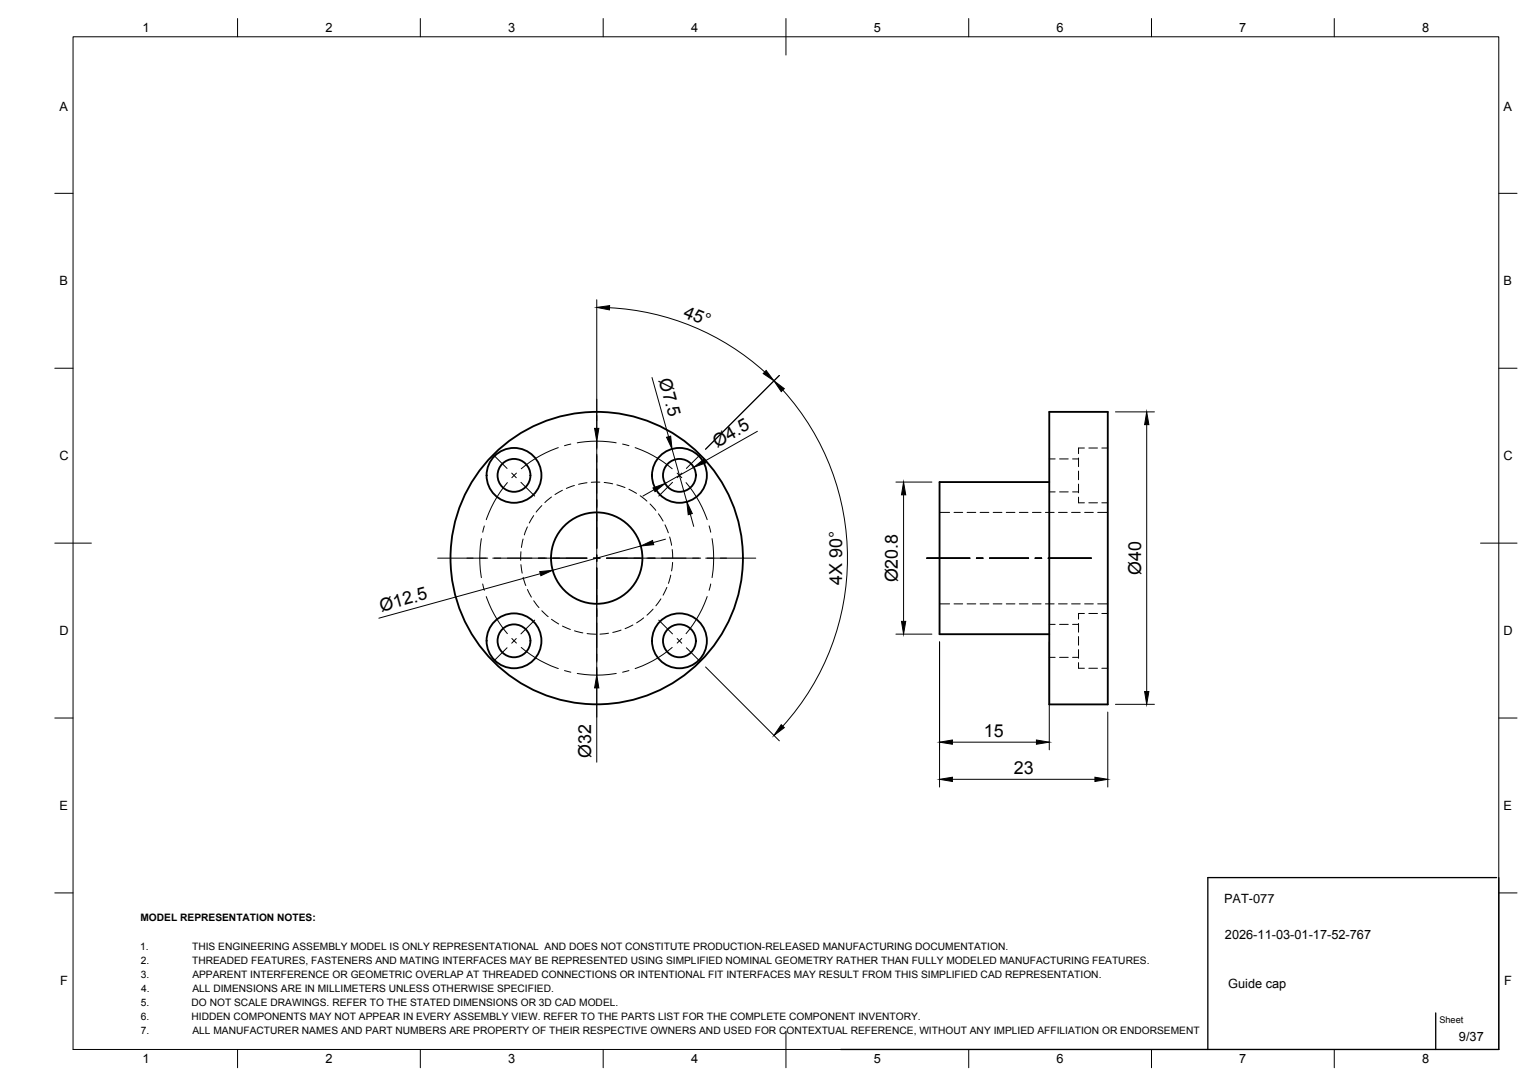
ISO-10303-21;
HEADER;
/* Generated by software containing ST-Developer
 * from STEP Tools, Inc. (www.steptools.com) 
 */

FILE_DESCRIPTION(
/* description */ ('Pallet stop with pneumatic fitting'),
/* implementation_level */ '2;1');

FILE_NAME(
/* name */ 'Guide cap.step',
/* time_stamp */ '2026-10-27T10:51:41-07:00',
/* author */ (''),
/* organization */ (''),
/* preprocessor_version */ 'ST-DEVELOPER v20.2',
/* originating_system */ 'Autodesk Translation Framework v15.17.0.0',
/* authorisation */ '');

FILE_SCHEMA (('AUTOMOTIVE_DESIGN { 1 0 10303 214 3 1 1 }'));
ENDSEC;

DATA;
#10=MECHANICAL_DESIGN_GEOMETRIC_PRESENTATION_REPRESENTATION('',(#361),#10265);
#297=SHAPE_REPRESENTATION_RELATIONSHIP('SRR','None',#10410,#329);
#329=ADVANCED_BREP_SHAPE_REPRESENTATION('',(#393),#10234);
#361=STYLED_ITEM('',(#10641),#393);
#393=MANIFOLD_SOLID_BREP('Body1',#5049);
#448=FACE_BOUND('',#1133,.T.);
#449=FACE_BOUND('',#1136,.T.);
#450=FACE_BOUND('',#1139,.T.);
#451=FACE_BOUND('',#1142,.T.);
#452=FACE_BOUND('',#1149,.T.);
#453=FACE_BOUND('',#1153,.T.);
#454=FACE_BOUND('',#1154,.T.);
#455=FACE_BOUND('',#1155,.T.);
#456=FACE_BOUND('',#1156,.T.);
#457=FACE_BOUND('',#1157,.T.);
#458=FACE_BOUND('',#1159,.T.);
#459=FACE_BOUND('',#1160,.T.);
#460=FACE_BOUND('',#1161,.T.);
#461=FACE_BOUND('',#1162,.T.);
#462=FACE_BOUND('',#1163,.T.);
#578=PLANE('',#5532);
#579=PLANE('',#5537);
#580=PLANE('',#5542);
#581=PLANE('',#5547);
#582=PLANE('',#5560);
#583=PLANE('',#5567);
#584=PLANE('',#5568);
#788=FACE_OUTER_BOUND('',#1131,.T.);
#789=FACE_OUTER_BOUND('',#1132,.T.);
#790=FACE_OUTER_BOUND('',#1134,.T.);
#791=FACE_OUTER_BOUND('',#1135,.T.);
#792=FACE_OUTER_BOUND('',#1137,.T.);
#793=FACE_OUTER_BOUND('',#1138,.T.);
#794=FACE_OUTER_BOUND('',#1140,.T.);
#795=FACE_OUTER_BOUND('',#1141,.T.);
#796=FACE_OUTER_BOUND('',#1143,.T.);
#797=FACE_OUTER_BOUND('',#1144,.T.);
#798=FACE_OUTER_BOUND('',#1145,.T.);
#799=FACE_OUTER_BOUND('',#1146,.T.);
#800=FACE_OUTER_BOUND('',#1147,.T.);
#801=FACE_OUTER_BOUND('',#1148,.T.);
#802=FACE_OUTER_BOUND('',#1150,.T.);
#803=FACE_OUTER_BOUND('',#1151,.T.);
#804=FACE_OUTER_BOUND('',#1152,.T.);
#805=FACE_OUTER_BOUND('',#1158,.T.);
#1131=EDGE_LOOP('',(#3620,#3621,#3622,#3623));
#1132=EDGE_LOOP('',(#3624));
#1133=EDGE_LOOP('',(#3625));
#1134=EDGE_LOOP('',(#3626,#3627,#3628,#3629));
#1135=EDGE_LOOP('',(#3630));
#1136=EDGE_LOOP('',(#3631));
#1137=EDGE_LOOP('',(#3632,#3633,#3634,#3635));
#1138=EDGE_LOOP('',(#3636));
#1139=EDGE_LOOP('',(#3637));
#1140=EDGE_LOOP('',(#3638,#3639,#3640,#3641));
#1141=EDGE_LOOP('',(#3642));
#1142=EDGE_LOOP('',(#3643));
#1143=EDGE_LOOP('',(#3644,#3645,#3646,#3647));
#1144=EDGE_LOOP('',(#3648,#3649,#3650,#3651));
#1145=EDGE_LOOP('',(#3652,#3653,#3654,#3655));
#1146=EDGE_LOOP('',(#3656,#3657,#3658,#3659));
#1147=EDGE_LOOP('',(#3660,#3661,#3662,#3663));
#1148=EDGE_LOOP('',(#3664));
#1149=EDGE_LOOP('',(#3665));
#1150=EDGE_LOOP('',(#3666,#3667,#3668,#3669));
#1151=EDGE_LOOP('',(#3670,#3671,#3672,#3673));
#1152=EDGE_LOOP('',(#3674));
#1153=EDGE_LOOP('',(#3675));
#1154=EDGE_LOOP('',(#3676));
#1155=EDGE_LOOP('',(#3677));
#1156=EDGE_LOOP('',(#3678));
#1157=EDGE_LOOP('',(#3679));
#1158=EDGE_LOOP('',(#3680));
#1159=EDGE_LOOP('',(#3681));
#1160=EDGE_LOOP('',(#3682));
#1161=EDGE_LOOP('',(#3683));
#1162=EDGE_LOOP('',(#3684));
#1163=EDGE_LOOP('',(#3685));
#1557=LINE('',#7976,#1892);
#1558=LINE('',#7985,#1893);
#1559=LINE('',#7994,#1894);
#1560=LINE('',#8003,#1895);
#1561=LINE('',#8011,#1896);
#1562=LINE('',#8015,#1897);
#1563=LINE('',#8019,#1898);
#1564=LINE('',#8023,#1899);
#1565=LINE('',#8028,#1900);
#1566=LINE('',#8036,#1901);
#1567=LINE('',#8041,#1902);
#1892=VECTOR('',#6354,0.375);
#1893=VECTOR('',#6365,0.375);
#1894=VECTOR('',#6376,0.375);
#1895=VECTOR('',#6387,0.375);
#1896=VECTOR('',#6398,0.225);
#1897=VECTOR('',#6403,0.225);
#1898=VECTOR('',#6408,0.225);
#1899=VECTOR('',#6413,0.225);
#1900=VECTOR('',#6418,1.04);
#1901=VECTOR('',#6429,0.625);
#1902=VECTOR('',#6434,2.);
#2198=CIRCLE('',#5530,0.375);
#2199=CIRCLE('',#5531,0.375);
#2200=CIRCLE('',#5533,0.225);
#2201=CIRCLE('',#5535,0.375);
#2202=CIRCLE('',#5536,0.375);
#2203=CIRCLE('',#5538,0.225);
#2204=CIRCLE('',#5540,0.375);
#2205=CIRCLE('',#5541,0.375);
#2206=CIRCLE('',#5543,0.225);
#2207=CIRCLE('',#5545,0.375);
#2208=CIRCLE('',#5546,0.375);
#2209=CIRCLE('',#5548,0.225);
#2210=CIRCLE('',#5550,0.225);
#2211=CIRCLE('',#5552,0.225);
#2212=CIRCLE('',#5554,0.225);
#2213=CIRCLE('',#5556,0.225);
#2214=CIRCLE('',#5558,1.04);
#2215=CIRCLE('',#5559,1.04);
#2216=CIRCLE('',#5561,0.625);
#2217=CIRCLE('',#5563,0.625);
#2218=CIRCLE('',#5565,2.);
#2219=CIRCLE('',#5566,2.);
#2477=VERTEX_POINT('',#7973);
#2478=VERTEX_POINT('',#7975);
#2479=VERTEX_POINT('',#7979);
#2480=VERTEX_POINT('',#7982);
#2481=VERTEX_POINT('',#7984);
#2482=VERTEX_POINT('',#7988);
#2483=VERTEX_POINT('',#7991);
#2484=VERTEX_POINT('',#7993);
#2485=VERTEX_POINT('',#7997);
#2486=VERTEX_POINT('',#8000);
#2487=VERTEX_POINT('',#8002);
#2488=VERTEX_POINT('',#8006);
#2489=VERTEX_POINT('',#8009);
#2490=VERTEX_POINT('',#8013);
#2491=VERTEX_POINT('',#8017);
#2492=VERTEX_POINT('',#8021);
#2493=VERTEX_POINT('',#8025);
#2494=VERTEX_POINT('',#8027);
#2495=VERTEX_POINT('',#8031);
#2496=VERTEX_POINT('',#8034);
#2497=VERTEX_POINT('',#8038);
#2498=VERTEX_POINT('',#8040);
#2909=EDGE_CURVE('',#2477,#2477,#2198,.T.);
#2910=EDGE_CURVE('',#2477,#2478,#1557,.T.);
#2911=EDGE_CURVE('',#2478,#2478,#2199,.T.);
#2912=EDGE_CURVE('',#2479,#2479,#2200,.T.);
#2913=EDGE_CURVE('',#2480,#2480,#2201,.T.);
#2914=EDGE_CURVE('',#2480,#2481,#1558,.T.);
#2915=EDGE_CURVE('',#2481,#2481,#2202,.T.);
#2916=EDGE_CURVE('',#2482,#2482,#2203,.T.);
#2917=EDGE_CURVE('',#2483,#2483,#2204,.T.);
#2918=EDGE_CURVE('',#2483,#2484,#1559,.T.);
#2919=EDGE_CURVE('',#2484,#2484,#2205,.T.);
#2920=EDGE_CURVE('',#2485,#2485,#2206,.T.);
#2921=EDGE_CURVE('',#2486,#2486,#2207,.T.);
#2922=EDGE_CURVE('',#2486,#2487,#1560,.T.);
#2923=EDGE_CURVE('',#2487,#2487,#2208,.T.);
#2924=EDGE_CURVE('',#2488,#2488,#2209,.T.);
#2925=EDGE_CURVE('',#2489,#2489,#2210,.T.);
#2926=EDGE_CURVE('',#2489,#2479,#1561,.T.);
#2927=EDGE_CURVE('',#2490,#2490,#2211,.T.);
#2928=EDGE_CURVE('',#2490,#2482,#1562,.T.);
#2929=EDGE_CURVE('',#2491,#2491,#2212,.T.);
#2930=EDGE_CURVE('',#2491,#2485,#1563,.T.);
#2931=EDGE_CURVE('',#2492,#2492,#2213,.T.);
#2932=EDGE_CURVE('',#2492,#2488,#1564,.T.);
#2933=EDGE_CURVE('',#2493,#2493,#2214,.T.);
#2934=EDGE_CURVE('',#2493,#2494,#1565,.T.);
#2935=EDGE_CURVE('',#2494,#2494,#2215,.T.);
#2936=EDGE_CURVE('',#2495,#2495,#2216,.T.);
#2937=EDGE_CURVE('',#2496,#2496,#2217,.T.);
#2938=EDGE_CURVE('',#2496,#2495,#1566,.T.);
#2939=EDGE_CURVE('',#2497,#2497,#2218,.T.);
#2940=EDGE_CURVE('',#2497,#2498,#1567,.T.);
#2941=EDGE_CURVE('',#2498,#2498,#2219,.T.);
#3620=ORIENTED_EDGE('',*,*,#2909,.F.);
#3621=ORIENTED_EDGE('',*,*,#2910,.T.);
#3622=ORIENTED_EDGE('',*,*,#2911,.F.);
#3623=ORIENTED_EDGE('',*,*,#2910,.F.);
#3624=ORIENTED_EDGE('',*,*,#2909,.T.);
#3625=ORIENTED_EDGE('',*,*,#2912,.F.);
#3626=ORIENTED_EDGE('',*,*,#2913,.F.);
#3627=ORIENTED_EDGE('',*,*,#2914,.T.);
#3628=ORIENTED_EDGE('',*,*,#2915,.F.);
#3629=ORIENTED_EDGE('',*,*,#2914,.F.);
#3630=ORIENTED_EDGE('',*,*,#2913,.T.);
#3631=ORIENTED_EDGE('',*,*,#2916,.F.);
#3632=ORIENTED_EDGE('',*,*,#2917,.F.);
#3633=ORIENTED_EDGE('',*,*,#2918,.T.);
#3634=ORIENTED_EDGE('',*,*,#2919,.F.);
#3635=ORIENTED_EDGE('',*,*,#2918,.F.);
#3636=ORIENTED_EDGE('',*,*,#2917,.T.);
#3637=ORIENTED_EDGE('',*,*,#2920,.F.);
#3638=ORIENTED_EDGE('',*,*,#2921,.F.);
#3639=ORIENTED_EDGE('',*,*,#2922,.T.);
#3640=ORIENTED_EDGE('',*,*,#2923,.F.);
#3641=ORIENTED_EDGE('',*,*,#2922,.F.);
#3642=ORIENTED_EDGE('',*,*,#2921,.T.);
#3643=ORIENTED_EDGE('',*,*,#2924,.F.);
#3644=ORIENTED_EDGE('',*,*,#2925,.F.);
#3645=ORIENTED_EDGE('',*,*,#2926,.T.);
#3646=ORIENTED_EDGE('',*,*,#2912,.T.);
#3647=ORIENTED_EDGE('',*,*,#2926,.F.);
#3648=ORIENTED_EDGE('',*,*,#2927,.F.);
#3649=ORIENTED_EDGE('',*,*,#2928,.T.);
#3650=ORIENTED_EDGE('',*,*,#2916,.T.);
#3651=ORIENTED_EDGE('',*,*,#2928,.F.);
#3652=ORIENTED_EDGE('',*,*,#2929,.F.);
#3653=ORIENTED_EDGE('',*,*,#2930,.T.);
#3654=ORIENTED_EDGE('',*,*,#2920,.T.);
#3655=ORIENTED_EDGE('',*,*,#2930,.F.);
#3656=ORIENTED_EDGE('',*,*,#2931,.F.);
#3657=ORIENTED_EDGE('',*,*,#2932,.T.);
#3658=ORIENTED_EDGE('',*,*,#2924,.T.);
#3659=ORIENTED_EDGE('',*,*,#2932,.F.);
#3660=ORIENTED_EDGE('',*,*,#2933,.F.);
#3661=ORIENTED_EDGE('',*,*,#2934,.T.);
#3662=ORIENTED_EDGE('',*,*,#2935,.T.);
#3663=ORIENTED_EDGE('',*,*,#2934,.F.);
#3664=ORIENTED_EDGE('',*,*,#2935,.F.);
#3665=ORIENTED_EDGE('',*,*,#2936,.F.);
#3666=ORIENTED_EDGE('',*,*,#2937,.F.);
#3667=ORIENTED_EDGE('',*,*,#2938,.T.);
#3668=ORIENTED_EDGE('',*,*,#2936,.T.);
#3669=ORIENTED_EDGE('',*,*,#2938,.F.);
#3670=ORIENTED_EDGE('',*,*,#2939,.F.);
#3671=ORIENTED_EDGE('',*,*,#2940,.T.);
#3672=ORIENTED_EDGE('',*,*,#2941,.T.);
#3673=ORIENTED_EDGE('',*,*,#2940,.F.);
#3674=ORIENTED_EDGE('',*,*,#2939,.T.);
#3675=ORIENTED_EDGE('',*,*,#2937,.T.);
#3676=ORIENTED_EDGE('',*,*,#2923,.T.);
#3677=ORIENTED_EDGE('',*,*,#2919,.T.);
#3678=ORIENTED_EDGE('',*,*,#2915,.T.);
#3679=ORIENTED_EDGE('',*,*,#2911,.T.);
#3680=ORIENTED_EDGE('',*,*,#2941,.F.);
#3681=ORIENTED_EDGE('',*,*,#2933,.T.);
#3682=ORIENTED_EDGE('',*,*,#2931,.T.);
#3683=ORIENTED_EDGE('',*,*,#2929,.T.);
#3684=ORIENTED_EDGE('',*,*,#2927,.T.);
#3685=ORIENTED_EDGE('',*,*,#2925,.T.);
#4641=CYLINDRICAL_SURFACE('',#5529,0.375);
#4642=CYLINDRICAL_SURFACE('',#5534,0.375);
#4643=CYLINDRICAL_SURFACE('',#5539,0.375);
#4644=CYLINDRICAL_SURFACE('',#5544,0.375);
#4645=CYLINDRICAL_SURFACE('',#5549,0.225);
#4646=CYLINDRICAL_SURFACE('',#5551,0.225);
#4647=CYLINDRICAL_SURFACE('',#5553,0.225);
#4648=CYLINDRICAL_SURFACE('',#5555,0.225);
#4649=CYLINDRICAL_SURFACE('',#5557,1.04);
#4650=CYLINDRICAL_SURFACE('',#5562,0.625);
#4651=CYLINDRICAL_SURFACE('',#5564,2.);
#4783=ADVANCED_FACE('',(#788),#4641,.F.);
#4784=ADVANCED_FACE('',(#789,#448),#578,.T.);
#4785=ADVANCED_FACE('',(#790),#4642,.F.);
#4786=ADVANCED_FACE('',(#791,#449),#579,.T.);
#4787=ADVANCED_FACE('',(#792),#4643,.F.);
#4788=ADVANCED_FACE('',(#793,#450),#580,.T.);
#4789=ADVANCED_FACE('',(#794),#4644,.F.);
#4790=ADVANCED_FACE('',(#795,#451),#581,.T.);
#4791=ADVANCED_FACE('',(#796),#4645,.F.);
#4792=ADVANCED_FACE('',(#797),#4646,.F.);
#4793=ADVANCED_FACE('',(#798),#4647,.F.);
#4794=ADVANCED_FACE('',(#799),#4648,.F.);
#4795=ADVANCED_FACE('',(#800),#4649,.T.);
#4796=ADVANCED_FACE('',(#801,#452),#582,.F.);
#4797=ADVANCED_FACE('',(#802),#4650,.F.);
#4798=ADVANCED_FACE('',(#803),#4651,.T.);
#4799=ADVANCED_FACE('',(#804,#453,#454,#455,#456,#457),#583,.T.);
#4800=ADVANCED_FACE('',(#805,#458,#459,#460,#461,#462),#584,.F.);
#5049=CLOSED_SHELL('',(#4783,#4784,#4785,#4786,#4787,#4788,#4789,#4790,
#4791,#4792,#4793,#4794,#4795,#4796,#4797,#4798,#4799,#4800));
#5528=AXIS2_PLACEMENT_3D('',#7971,#6348,#6349);
#5529=AXIS2_PLACEMENT_3D('',#7972,#6350,#6351);
#5530=AXIS2_PLACEMENT_3D('',#7974,#6352,#6353);
#5531=AXIS2_PLACEMENT_3D('',#7977,#6355,#6356);
#5532=AXIS2_PLACEMENT_3D('',#7978,#6357,#6358);
#5533=AXIS2_PLACEMENT_3D('',#7980,#6359,#6360);
#5534=AXIS2_PLACEMENT_3D('',#7981,#6361,#6362);
#5535=AXIS2_PLACEMENT_3D('',#7983,#6363,#6364);
#5536=AXIS2_PLACEMENT_3D('',#7986,#6366,#6367);
#5537=AXIS2_PLACEMENT_3D('',#7987,#6368,#6369);
#5538=AXIS2_PLACEMENT_3D('',#7989,#6370,#6371);
#5539=AXIS2_PLACEMENT_3D('',#7990,#6372,#6373);
#5540=AXIS2_PLACEMENT_3D('',#7992,#6374,#6375);
#5541=AXIS2_PLACEMENT_3D('',#7995,#6377,#6378);
#5542=AXIS2_PLACEMENT_3D('',#7996,#6379,#6380);
#5543=AXIS2_PLACEMENT_3D('',#7998,#6381,#6382);
#5544=AXIS2_PLACEMENT_3D('',#7999,#6383,#6384);
#5545=AXIS2_PLACEMENT_3D('',#8001,#6385,#6386);
#5546=AXIS2_PLACEMENT_3D('',#8004,#6388,#6389);
#5547=AXIS2_PLACEMENT_3D('',#8005,#6390,#6391);
#5548=AXIS2_PLACEMENT_3D('',#8007,#6392,#6393);
#5549=AXIS2_PLACEMENT_3D('',#8008,#6394,#6395);
#5550=AXIS2_PLACEMENT_3D('',#8010,#6396,#6397);
#5551=AXIS2_PLACEMENT_3D('',#8012,#6399,#6400);
#5552=AXIS2_PLACEMENT_3D('',#8014,#6401,#6402);
#5553=AXIS2_PLACEMENT_3D('',#8016,#6404,#6405);
#5554=AXIS2_PLACEMENT_3D('',#8018,#6406,#6407);
#5555=AXIS2_PLACEMENT_3D('',#8020,#6409,#6410);
#5556=AXIS2_PLACEMENT_3D('',#8022,#6411,#6412);
#5557=AXIS2_PLACEMENT_3D('',#8024,#6414,#6415);
#5558=AXIS2_PLACEMENT_3D('',#8026,#6416,#6417);
#5559=AXIS2_PLACEMENT_3D('',#8029,#6419,#6420);
#5560=AXIS2_PLACEMENT_3D('',#8030,#6421,#6422);
#5561=AXIS2_PLACEMENT_3D('',#8032,#6423,#6424);
#5562=AXIS2_PLACEMENT_3D('',#8033,#6425,#6426);
#5563=AXIS2_PLACEMENT_3D('',#8035,#6427,#6428);
#5564=AXIS2_PLACEMENT_3D('',#8037,#6430,#6431);
#5565=AXIS2_PLACEMENT_3D('',#8039,#6432,#6433);
#5566=AXIS2_PLACEMENT_3D('',#8042,#6435,#6436);
#5567=AXIS2_PLACEMENT_3D('',#8043,#6437,#6438);
#5568=AXIS2_PLACEMENT_3D('',#8044,#6439,#6440);
#6348=DIRECTION('axis',(0.,0.,1.));
#6349=DIRECTION('refdir',(1.,0.,0.));
#6350=DIRECTION('center_axis',(0.,0.,1.));
#6351=DIRECTION('ref_axis',(1.,0.,0.));
#6352=DIRECTION('center_axis',(0.,0.,1.));
#6353=DIRECTION('ref_axis',(1.,0.,0.));
#6354=DIRECTION('',(0.,0.,1.));
#6355=DIRECTION('center_axis',(0.,0.,-1.));
#6356=DIRECTION('ref_axis',(1.,0.,0.));
#6357=DIRECTION('center_axis',(0.,0.,1.));
#6358=DIRECTION('ref_axis',(1.,0.,0.));
#6359=DIRECTION('center_axis',(0.,0.,1.));
#6360=DIRECTION('ref_axis',(1.,0.,0.));
#6361=DIRECTION('center_axis',(0.,0.,1.));
#6362=DIRECTION('ref_axis',(1.,0.,0.));
#6363=DIRECTION('center_axis',(0.,0.,1.));
#6364=DIRECTION('ref_axis',(1.,0.,0.));
#6365=DIRECTION('',(0.,0.,1.));
#6366=DIRECTION('center_axis',(0.,0.,-1.));
#6367=DIRECTION('ref_axis',(1.,0.,0.));
#6368=DIRECTION('center_axis',(0.,0.,1.));
#6369=DIRECTION('ref_axis',(1.,0.,0.));
#6370=DIRECTION('center_axis',(0.,0.,1.));
#6371=DIRECTION('ref_axis',(1.,0.,0.));
#6372=DIRECTION('center_axis',(0.,0.,1.));
#6373=DIRECTION('ref_axis',(1.,0.,0.));
#6374=DIRECTION('center_axis',(0.,0.,1.));
#6375=DIRECTION('ref_axis',(1.,0.,0.));
#6376=DIRECTION('',(0.,0.,1.));
#6377=DIRECTION('center_axis',(0.,0.,-1.));
#6378=DIRECTION('ref_axis',(1.,0.,0.));
#6379=DIRECTION('center_axis',(0.,0.,1.));
#6380=DIRECTION('ref_axis',(1.,0.,0.));
#6381=DIRECTION('center_axis',(0.,0.,1.));
#6382=DIRECTION('ref_axis',(1.,0.,0.));
#6383=DIRECTION('center_axis',(0.,0.,1.));
#6384=DIRECTION('ref_axis',(1.,0.,0.));
#6385=DIRECTION('center_axis',(0.,0.,1.));
#6386=DIRECTION('ref_axis',(1.,0.,0.));
#6387=DIRECTION('',(0.,0.,1.));
#6388=DIRECTION('center_axis',(0.,0.,-1.));
#6389=DIRECTION('ref_axis',(1.,0.,0.));
#6390=DIRECTION('center_axis',(0.,0.,1.));
#6391=DIRECTION('ref_axis',(1.,0.,0.));
#6392=DIRECTION('center_axis',(0.,0.,1.));
#6393=DIRECTION('ref_axis',(1.,0.,0.));
#6394=DIRECTION('center_axis',(0.,0.,1.));
#6395=DIRECTION('ref_axis',(1.,0.,0.));
#6396=DIRECTION('center_axis',(0.,0.,1.));
#6397=DIRECTION('ref_axis',(1.,0.,0.));
#6398=DIRECTION('',(0.,0.,1.));
#6399=DIRECTION('center_axis',(0.,0.,1.));
#6400=DIRECTION('ref_axis',(1.,0.,0.));
#6401=DIRECTION('center_axis',(0.,0.,1.));
#6402=DIRECTION('ref_axis',(1.,0.,0.));
#6403=DIRECTION('',(0.,0.,1.));
#6404=DIRECTION('center_axis',(0.,0.,1.));
#6405=DIRECTION('ref_axis',(1.,0.,0.));
#6406=DIRECTION('center_axis',(0.,0.,1.));
#6407=DIRECTION('ref_axis',(1.,0.,0.));
#6408=DIRECTION('',(0.,0.,1.));
#6409=DIRECTION('center_axis',(0.,0.,1.));
#6410=DIRECTION('ref_axis',(1.,0.,0.));
#6411=DIRECTION('center_axis',(0.,0.,1.));
#6412=DIRECTION('ref_axis',(1.,0.,0.));
#6413=DIRECTION('',(0.,0.,1.));
#6414=DIRECTION('center_axis',(0.,0.,1.));
#6415=DIRECTION('ref_axis',(1.,0.,0.));
#6416=DIRECTION('center_axis',(0.,0.,1.));
#6417=DIRECTION('ref_axis',(1.,0.,0.));
#6418=DIRECTION('',(0.,0.,-1.));
#6419=DIRECTION('center_axis',(0.,0.,1.));
#6420=DIRECTION('ref_axis',(1.,0.,0.));
#6421=DIRECTION('center_axis',(0.,0.,1.));
#6422=DIRECTION('ref_axis',(1.,0.,0.));
#6423=DIRECTION('center_axis',(0.,0.,-1.));
#6424=DIRECTION('ref_axis',(1.,0.,0.));
#6425=DIRECTION('center_axis',(0.,0.,1.));
#6426=DIRECTION('ref_axis',(1.,0.,0.));
#6427=DIRECTION('center_axis',(0.,0.,-1.));
#6428=DIRECTION('ref_axis',(1.,0.,0.));
#6429=DIRECTION('',(0.,0.,-1.));
#6430=DIRECTION('center_axis',(0.,0.,1.));
#6431=DIRECTION('ref_axis',(1.,0.,0.));
#6432=DIRECTION('center_axis',(0.,0.,1.));
#6433=DIRECTION('ref_axis',(1.,0.,0.));
#6434=DIRECTION('',(0.,0.,-1.));
#6435=DIRECTION('center_axis',(0.,0.,1.));
#6436=DIRECTION('ref_axis',(1.,0.,0.));
#6437=DIRECTION('center_axis',(0.,0.,1.));
#6438=DIRECTION('ref_axis',(1.,0.,0.));
#6439=DIRECTION('center_axis',(0.,0.,1.));
#6440=DIRECTION('ref_axis',(1.,0.,0.));
#7971=CARTESIAN_POINT('',(0.,0.,0.));
#7972=CARTESIAN_POINT('Origin',(-1.13137084989848,-1.13137084989848,8.4));
#7973=CARTESIAN_POINT('',(-1.50637084989848,-1.13137084989848,8.4));
#7974=CARTESIAN_POINT('Origin',(-1.13137084989848,-1.13137084989848,8.4));
#7975=CARTESIAN_POINT('',(-1.50637084989848,-1.13137084989848,8.8));
#7976=CARTESIAN_POINT('',(-1.50637084989848,-1.13137084989848,8.4));
#7977=CARTESIAN_POINT('Origin',(-1.13137084989848,-1.13137084989848,8.8));
#7978=CARTESIAN_POINT('Origin',(-1.13137084989848,-1.13137084989848,8.4));
#7979=CARTESIAN_POINT('',(-1.35637084989848,-1.13137084989848,8.4));
#7980=CARTESIAN_POINT('Origin',(-1.13137084989848,-1.13137084989848,8.4));
#7981=CARTESIAN_POINT('Origin',(-1.13137084989848,1.13137084989848,8.4));
#7982=CARTESIAN_POINT('',(-1.50637084989848,1.13137084989848,8.4));
#7983=CARTESIAN_POINT('Origin',(-1.13137084989848,1.13137084989848,8.4));
#7984=CARTESIAN_POINT('',(-1.50637084989848,1.13137084989848,8.8));
#7985=CARTESIAN_POINT('',(-1.50637084989848,1.13137084989848,8.4));
#7986=CARTESIAN_POINT('Origin',(-1.13137084989848,1.13137084989848,8.8));
#7987=CARTESIAN_POINT('Origin',(-1.13137084989848,1.13137084989848,8.4));
#7988=CARTESIAN_POINT('',(-1.35637084989848,1.13137084989848,8.4));
#7989=CARTESIAN_POINT('Origin',(-1.13137084989848,1.13137084989848,8.4));
#7990=CARTESIAN_POINT('Origin',(1.13137084989848,1.13137084989848,8.4));
#7991=CARTESIAN_POINT('',(0.756370849898476,1.13137084989848,8.4));
#7992=CARTESIAN_POINT('Origin',(1.13137084989848,1.13137084989848,8.4));
#7993=CARTESIAN_POINT('',(0.756370849898476,1.13137084989848,8.8));
#7994=CARTESIAN_POINT('',(0.756370849898476,1.13137084989848,8.4));
#7995=CARTESIAN_POINT('Origin',(1.13137084989848,1.13137084989848,8.8));
#7996=CARTESIAN_POINT('Origin',(1.13137084989848,1.13137084989848,8.4));
#7997=CARTESIAN_POINT('',(0.906370849898476,1.13137084989848,8.4));
#7998=CARTESIAN_POINT('Origin',(1.13137084989848,1.13137084989848,8.4));
#7999=CARTESIAN_POINT('Origin',(1.13137084989848,-1.13137084989848,8.4));
#8000=CARTESIAN_POINT('',(0.756370849898476,-1.13137084989848,8.4));
#8001=CARTESIAN_POINT('Origin',(1.13137084989848,-1.13137084989848,8.4));
#8002=CARTESIAN_POINT('',(0.756370849898476,-1.13137084989848,8.8));
#8003=CARTESIAN_POINT('',(0.756370849898476,-1.13137084989848,8.4));
#8004=CARTESIAN_POINT('Origin',(1.13137084989848,-1.13137084989848,8.8));
#8005=CARTESIAN_POINT('Origin',(1.13137084989848,-1.13137084989848,8.4));
#8006=CARTESIAN_POINT('',(0.906370849898476,-1.13137084989848,8.4));
#8007=CARTESIAN_POINT('Origin',(1.13137084989848,-1.13137084989848,8.4));
#8008=CARTESIAN_POINT('Origin',(-1.13137084989848,-1.13137084989848,7.9));
#8009=CARTESIAN_POINT('',(-1.35637084989848,-1.13137084989848,8.));
#8010=CARTESIAN_POINT('Origin',(-1.13137084989848,-1.13137084989848,8.));
#8011=CARTESIAN_POINT('',(-1.35637084989848,-1.13137084989848,7.9));
#8012=CARTESIAN_POINT('Origin',(-1.13137084989848,1.13137084989848,7.9));
#8013=CARTESIAN_POINT('',(-1.35637084989848,1.13137084989848,8.));
#8014=CARTESIAN_POINT('Origin',(-1.13137084989848,1.13137084989848,8.));
#8015=CARTESIAN_POINT('',(-1.35637084989848,1.13137084989848,7.9));
#8016=CARTESIAN_POINT('Origin',(1.13137084989848,1.13137084989848,7.9));
#8017=CARTESIAN_POINT('',(0.906370849898476,1.13137084989848,8.));
#8018=CARTESIAN_POINT('Origin',(1.13137084989848,1.13137084989848,8.));
#8019=CARTESIAN_POINT('',(0.906370849898476,1.13137084989848,7.9));
#8020=CARTESIAN_POINT('Origin',(1.13137084989848,-1.13137084989848,7.9));
#8021=CARTESIAN_POINT('',(0.906370849898476,-1.13137084989848,8.));
#8022=CARTESIAN_POINT('Origin',(1.13137084989848,-1.13137084989848,8.));
#8023=CARTESIAN_POINT('',(0.906370849898476,-1.13137084989848,7.9));
#8024=CARTESIAN_POINT('Origin',(0.,0.,6.5));
#8025=CARTESIAN_POINT('',(-1.04,-1.27363267111325E-16,8.));
#8026=CARTESIAN_POINT('Origin',(0.,0.,8.));
#8027=CARTESIAN_POINT('',(-1.04,-1.27363267111325E-16,6.5));
#8028=CARTESIAN_POINT('',(-1.04,-1.27363267111325E-16,6.5));
#8029=CARTESIAN_POINT('Origin',(0.,0.,6.5));
#8030=CARTESIAN_POINT('Origin',(0.,0.,6.5));
#8031=CARTESIAN_POINT('',(-0.625,-7.65404249467096E-17,6.5));
#8032=CARTESIAN_POINT('Origin',(0.,0.,6.5));
#8033=CARTESIAN_POINT('Origin',(0.,0.,8.));
#8034=CARTESIAN_POINT('',(-0.625,-7.65404249467096E-17,8.8));
#8035=CARTESIAN_POINT('Origin',(0.,0.,8.8));
#8036=CARTESIAN_POINT('',(-0.625,-7.65404249467096E-17,8.));
#8037=CARTESIAN_POINT('Origin',(0.,0.,8.));
#8038=CARTESIAN_POINT('',(-2.,-2.44929359829471E-16,8.8));
#8039=CARTESIAN_POINT('Origin',(0.,0.,8.8));
#8040=CARTESIAN_POINT('',(-2.,-2.44929359829471E-16,8.));
#8041=CARTESIAN_POINT('',(-2.,-2.44929359829471E-16,8.));
#8042=CARTESIAN_POINT('Origin',(0.,0.,8.));
#8043=CARTESIAN_POINT('Origin',(0.,0.,8.8));
#8044=CARTESIAN_POINT('Origin',(0.,0.,8.));
#10196=UNCERTAINTY_MEASURE_WITH_UNIT(LENGTH_MEASURE(0.001),#10266,
'DISTANCE_ACCURACY_VALUE',
'Maximum model space distance between geometric entities at asserted c
onnectivities');
#10227=UNCERTAINTY_MEASURE_WITH_UNIT(LENGTH_MEASURE(0.001),#10266,
'DISTANCE_ACCURACY_VALUE',
'Maximum model space distance between geometric entities at asserted c
onnectivities');
#10234=(
GEOMETRIC_REPRESENTATION_CONTEXT(3)
GLOBAL_UNCERTAINTY_ASSIGNED_CONTEXT((#10196))
GLOBAL_UNIT_ASSIGNED_CONTEXT((#10266,#10268,#10269))
REPRESENTATION_CONTEXT('','3D')
);
#10265=(
GEOMETRIC_REPRESENTATION_CONTEXT(3)
GLOBAL_UNCERTAINTY_ASSIGNED_CONTEXT((#10227))
GLOBAL_UNIT_ASSIGNED_CONTEXT((#10266,#10268,#10269))
REPRESENTATION_CONTEXT('','3D')
);
#10266=(
LENGTH_UNIT()
NAMED_UNIT(*)
SI_UNIT(.CENTI.,.METRE.)
);
#10268=(
NAMED_UNIT(*)
PLANE_ANGLE_UNIT()
SI_UNIT($,.RADIAN.)
);
#10269=(
NAMED_UNIT(*)
SI_UNIT($,.STERADIAN.)
SOLID_ANGLE_UNIT()
);
#10276=SHAPE_DEFINITION_REPRESENTATION(#10313,#10410);
#10313=PRODUCT_DEFINITION_SHAPE('',$,#10448);
#10410=SHAPE_REPRESENTATION('',(#5528),#10234);
#10441=PRODUCT_DEFINITION_CONTEXT('part definition',#10554,'design');
#10448=PRODUCT_DEFINITION('Guide cap','Guide cap',#10485,#10441);
#10485=PRODUCT_DEFINITION_FORMATION('',$,#10562);
#10554=APPLICATION_CONTEXT(
'Core Data for Automotive Mechanical Design Process');
#10555=PRODUCT_CONTEXT('part definition',#10554,'mechanical');
#10562=PRODUCT('Guide cap','Guide cap','Guide cap',(#10555));
#10635=COLOUR_RGB('Light Blue',0.38,0.62,0.78);
#10636=FILL_AREA_STYLE_COLOUR('',#10635);
#10637=FILL_AREA_STYLE('',(#10636));
#10638=SURFACE_STYLE_FILL_AREA(#10637);
#10639=SURFACE_SIDE_STYLE('',(#10638));
#10640=SURFACE_STYLE_USAGE(.BOTH.,#10639);
#10641=PRESENTATION_STYLE_ASSIGNMENT((#10640));
ENDSEC;
END-ISO-10303-21;
